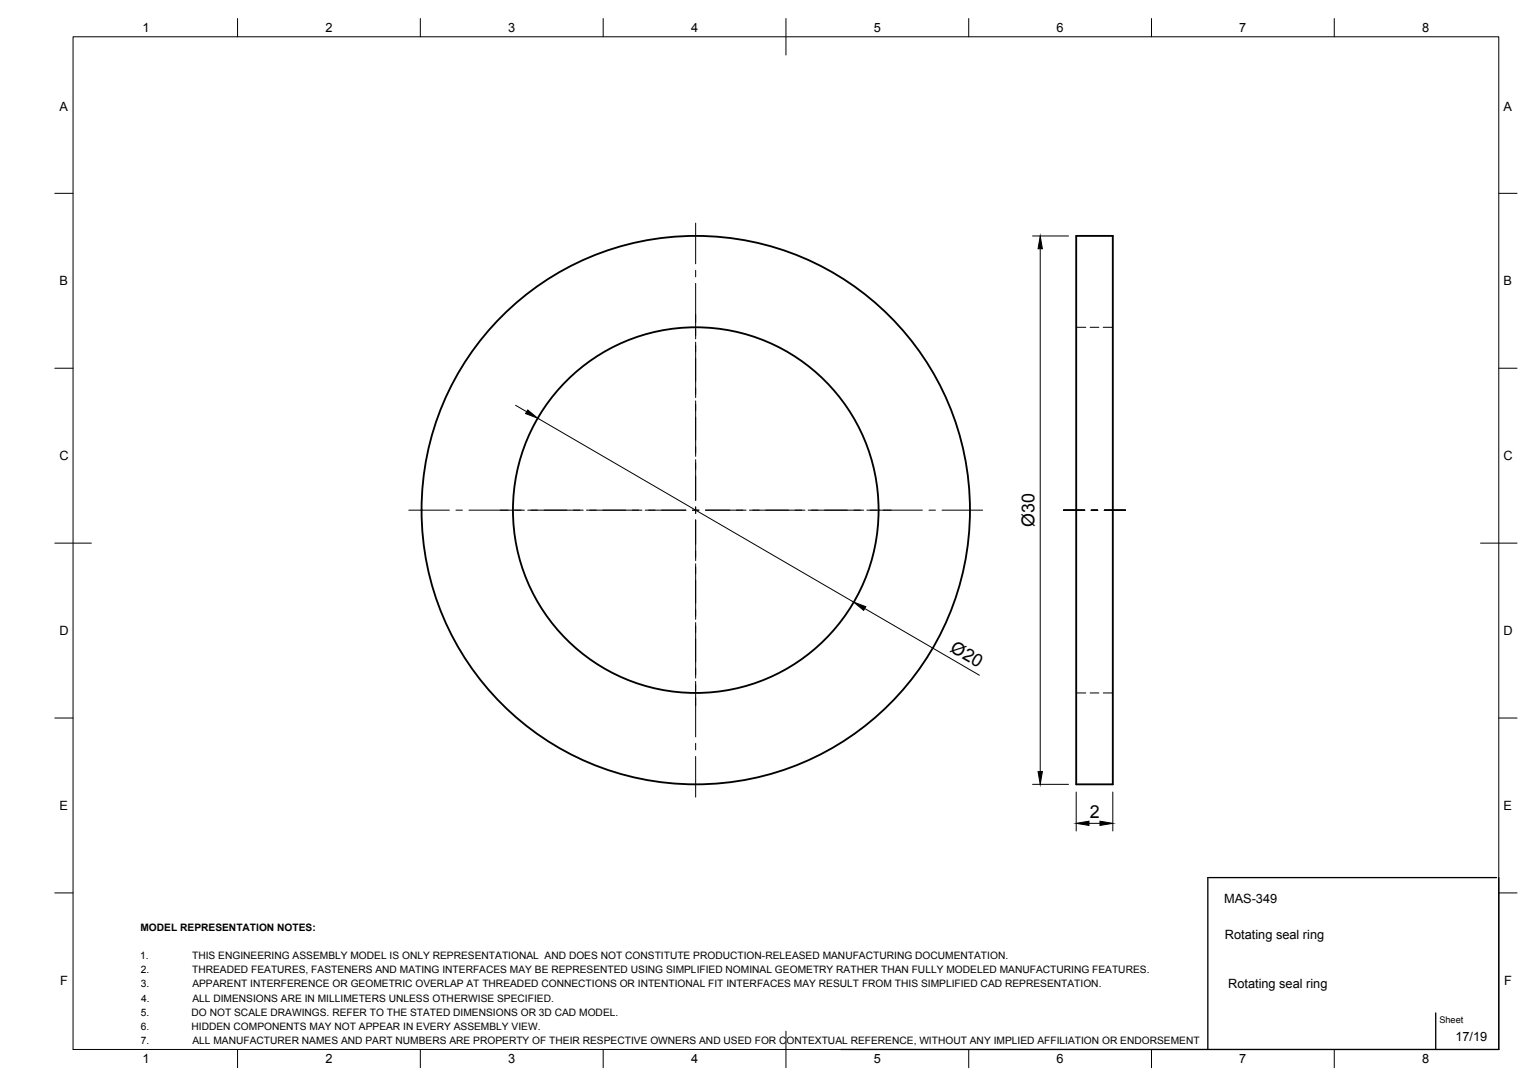
ISO-10303-21;
HEADER;
/* Generated by software containing ST-Developer
 * from STEP Tools, Inc. (www.steptools.com) 
 */

FILE_DESCRIPTION(
/* description */ ('Independent two-stage semi-open centrifugal-pump CAD. Shared impeller
s, open-machinable return casings, removable diaphragms, bronze wear/j
ournal rings, volume-preserving seal instances, retained keyed shaft, 
opposed mechanical face rings and partly threaded tie hardware. Native
 shaft rotation. Geometric topology/clearance only; flow/head/efficien
cy, pressure, cavitation, balance, preload, face loading and secondary
 seal fits/bonds, material/thermal/tolerance selection and life unassi
gned. External drive, coupling, anchors and piping bolts omitted.'),
/* implementation_level */ '2;1');

FILE_NAME(
/* name */ 'Rotating seal ring.step',
/* time_stamp */ '2026-11-08T18:06:32-08:00',
/* author */ (''),
/* organization */ (''),
/* preprocessor_version */ 'ST-DEVELOPER v20.2',
/* originating_system */ 'Autodesk Translation Framework v15.17.0.0',
/* authorisation */ '');

FILE_SCHEMA (('AUTOMOTIVE_DESIGN { 1 0 10303 214 3 1 1 }'));
ENDSEC;

DATA;
#10=MECHANICAL_DESIGN_GEOMETRIC_PRESENTATION_REPRESENTATION('',(#407),#16687);
#369=SHAPE_REPRESENTATION_RELATIONSHIP('SRR','None',#16778,#388);
#388=ADVANCED_BREP_SHAPE_REPRESENTATION('',(#426),#16682);
#407=STYLED_ITEM('',(#16877),#426);
#426=MANIFOLD_SOLID_BREP('Body1',#6126);
#545=FACE_BOUND('',#1448,.T.);
#546=FACE_BOUND('',#1450,.T.);
#665=PLANE('',#6887);
#666=PLANE('',#6888);
#984=FACE_OUTER_BOUND('',#1445,.T.);
#985=FACE_OUTER_BOUND('',#1446,.T.);
#986=FACE_OUTER_BOUND('',#1447,.T.);
#987=FACE_OUTER_BOUND('',#1449,.T.);
#1445=EDGE_LOOP('',(#5341,#5342,#5343,#5344));
#1446=EDGE_LOOP('',(#5345,#5346,#5347,#5348));
#1447=EDGE_LOOP('',(#5349));
#1448=EDGE_LOOP('',(#5350));
#1449=EDGE_LOOP('',(#5351));
#1450=EDGE_LOOP('',(#5352));
#1822=LINE('',#15207,#2191);
#1823=LINE('',#15213,#2192);
#2191=VECTOR('',#8392,1.);
#2192=VECTOR('',#8399,1.5);
#2474=CIRCLE('',#6882,1.);
#2475=CIRCLE('',#6883,1.);
#2476=CIRCLE('',#6885,1.5);
#2477=CIRCLE('',#6886,1.5);
#2981=VERTEX_POINT('',#15204);
#2982=VERTEX_POINT('',#15206);
#2983=VERTEX_POINT('',#15210);
#2984=VERTEX_POINT('',#15212);
#3780=EDGE_CURVE('',#2981,#2981,#2474,.T.);
#3781=EDGE_CURVE('',#2981,#2982,#1822,.T.);
#3782=EDGE_CURVE('',#2982,#2982,#2475,.T.);
#3783=EDGE_CURVE('',#2983,#2983,#2476,.T.);
#3784=EDGE_CURVE('',#2983,#2984,#1823,.T.);
#3785=EDGE_CURVE('',#2984,#2984,#2477,.T.);
#5341=ORIENTED_EDGE('',*,*,#3780,.F.);
#5342=ORIENTED_EDGE('',*,*,#3781,.T.);
#5343=ORIENTED_EDGE('',*,*,#3782,.T.);
#5344=ORIENTED_EDGE('',*,*,#3781,.F.);
#5345=ORIENTED_EDGE('',*,*,#3783,.F.);
#5346=ORIENTED_EDGE('',*,*,#3784,.T.);
#5347=ORIENTED_EDGE('',*,*,#3785,.T.);
#5348=ORIENTED_EDGE('',*,*,#3784,.F.);
#5349=ORIENTED_EDGE('',*,*,#3783,.T.);
#5350=ORIENTED_EDGE('',*,*,#3780,.T.);
#5351=ORIENTED_EDGE('',*,*,#3785,.F.);
#5352=ORIENTED_EDGE('',*,*,#3782,.F.);
#5740=CYLINDRICAL_SURFACE('',#6881,1.);
#5741=CYLINDRICAL_SURFACE('',#6884,1.5);
#6063=ADVANCED_FACE('',(#984),#5740,.F.);
#6064=ADVANCED_FACE('',(#985),#5741,.T.);
#6065=ADVANCED_FACE('',(#986,#545),#665,.T.);
#6066=ADVANCED_FACE('',(#987,#546),#666,.F.);
#6126=CLOSED_SHELL('',(#6063,#6064,#6065,#6066));
#6880=AXIS2_PLACEMENT_3D('',#15202,#8386,#8387);
#6881=AXIS2_PLACEMENT_3D('',#15203,#8388,#8389);
#6882=AXIS2_PLACEMENT_3D('',#15205,#8390,#8391);
#6883=AXIS2_PLACEMENT_3D('',#15208,#8393,#8394);
#6884=AXIS2_PLACEMENT_3D('',#15209,#8395,#8396);
#6885=AXIS2_PLACEMENT_3D('',#15211,#8397,#8398);
#6886=AXIS2_PLACEMENT_3D('',#15214,#8400,#8401);
#6887=AXIS2_PLACEMENT_3D('',#15215,#8402,#8403);
#6888=AXIS2_PLACEMENT_3D('',#15216,#8404,#8405);
#8386=DIRECTION('axis',(0.,0.,1.));
#8387=DIRECTION('refdir',(1.,0.,0.));
#8388=DIRECTION('center_axis',(0.,0.,1.));
#8389=DIRECTION('ref_axis',(1.,0.,0.));
#8390=DIRECTION('center_axis',(0.,0.,-1.));
#8391=DIRECTION('ref_axis',(1.,0.,0.));
#8392=DIRECTION('',(0.,0.,-1.));
#8393=DIRECTION('center_axis',(0.,0.,-1.));
#8394=DIRECTION('ref_axis',(1.,0.,0.));
#8395=DIRECTION('center_axis',(0.,0.,1.));
#8396=DIRECTION('ref_axis',(1.,0.,0.));
#8397=DIRECTION('center_axis',(0.,0.,1.));
#8398=DIRECTION('ref_axis',(1.,0.,0.));
#8399=DIRECTION('',(0.,0.,-1.));
#8400=DIRECTION('center_axis',(0.,0.,1.));
#8401=DIRECTION('ref_axis',(1.,0.,0.));
#8402=DIRECTION('center_axis',(0.,0.,1.));
#8403=DIRECTION('ref_axis',(1.,0.,0.));
#8404=DIRECTION('center_axis',(0.,0.,1.));
#8405=DIRECTION('ref_axis',(1.,0.,0.));
#15202=CARTESIAN_POINT('',(0.,0.,0.));
#15203=CARTESIAN_POINT('Origin',(0.,0.,11.2));
#15204=CARTESIAN_POINT('',(-1.,-1.22464679914735E-16,11.4));
#15205=CARTESIAN_POINT('Origin',(0.,0.,11.4));
#15206=CARTESIAN_POINT('',(-1.,-1.22464679914735E-16,11.2));
#15207=CARTESIAN_POINT('',(-1.,-1.22464679914735E-16,11.2));
#15208=CARTESIAN_POINT('Origin',(0.,0.,11.2));
#15209=CARTESIAN_POINT('Origin',(0.,0.,11.2));
#15210=CARTESIAN_POINT('',(-1.5,-1.83697019872103E-16,11.4));
#15211=CARTESIAN_POINT('Origin',(0.,0.,11.4));
#15212=CARTESIAN_POINT('',(-1.5,-1.83697019872103E-16,11.2));
#15213=CARTESIAN_POINT('',(-1.5,-1.83697019872103E-16,11.2));
#15214=CARTESIAN_POINT('Origin',(0.,0.,11.2));
#15215=CARTESIAN_POINT('Origin',(0.,0.,11.4));
#15216=CARTESIAN_POINT('Origin',(0.,0.,11.2));
#16661=UNCERTAINTY_MEASURE_WITH_UNIT(LENGTH_MEASURE(0.001),#16688,
'DISTANCE_ACCURACY_VALUE',
'Maximum model space distance between geometric entities at asserted c
onnectivities');
#16666=UNCERTAINTY_MEASURE_WITH_UNIT(LENGTH_MEASURE(0.001),#16688,
'DISTANCE_ACCURACY_VALUE',
'Maximum model space distance between geometric entities at asserted c
onnectivities');
#16682=(
GEOMETRIC_REPRESENTATION_CONTEXT(3)
GLOBAL_UNCERTAINTY_ASSIGNED_CONTEXT((#16661))
GLOBAL_UNIT_ASSIGNED_CONTEXT((#16688,#16690,#16691))
REPRESENTATION_CONTEXT('','3D')
);
#16687=(
GEOMETRIC_REPRESENTATION_CONTEXT(3)
GLOBAL_UNCERTAINTY_ASSIGNED_CONTEXT((#16666))
GLOBAL_UNIT_ASSIGNED_CONTEXT((#16688,#16690,#16691))
REPRESENTATION_CONTEXT('','3D')
);
#16688=(
LENGTH_UNIT()
NAMED_UNIT(*)
SI_UNIT(.CENTI.,.METRE.)
);
#16690=(
NAMED_UNIT(*)
PLANE_ANGLE_UNIT()
SI_UNIT($,.RADIAN.)
);
#16691=(
NAMED_UNIT(*)
SI_UNIT($,.STERADIAN.)
SOLID_ANGLE_UNIT()
);
#16707=SHAPE_DEFINITION_REPRESENTATION(#16727,#16778);
#16727=PRODUCT_DEFINITION_SHAPE('',$,#16799);
#16778=SHAPE_REPRESENTATION('',(#6880),#16682);
#16783=PRODUCT_DEFINITION_CONTEXT('part definition',#16845,'design');
#16799=PRODUCT_DEFINITION('Rotating seal ring','Rotating seal ring',#16819,
#16783);
#16819=PRODUCT_DEFINITION_FORMATION('',$,#16862);
#16845=APPLICATION_CONTEXT(
'Core Data for Automotive Mechanical Design Process');
#16846=PRODUCT_CONTEXT('part definition',#16845,'mechanical');
#16862=PRODUCT('Rotating seal ring','Rotating seal ring',$,(#16846));
#16877=PRESENTATION_STYLE_ASSIGNMENT((#16892));
#16892=SURFACE_STYLE_USAGE(.BOTH.,#16907);
#16907=SURFACE_SIDE_STYLE('',(#16922));
#16922=SURFACE_STYLE_FILL_AREA(#16937);
#16937=FILL_AREA_STYLE('Face seal light gray',(#16952));
#16952=FILL_AREA_STYLE_COLOUR('Face seal light gray',#16967);
#16967=COLOUR_RGB('Face seal light gray',0.725490196078431,0.752941176470588,
0.792156862745098);
ENDSEC;
END-ISO-10303-21;
